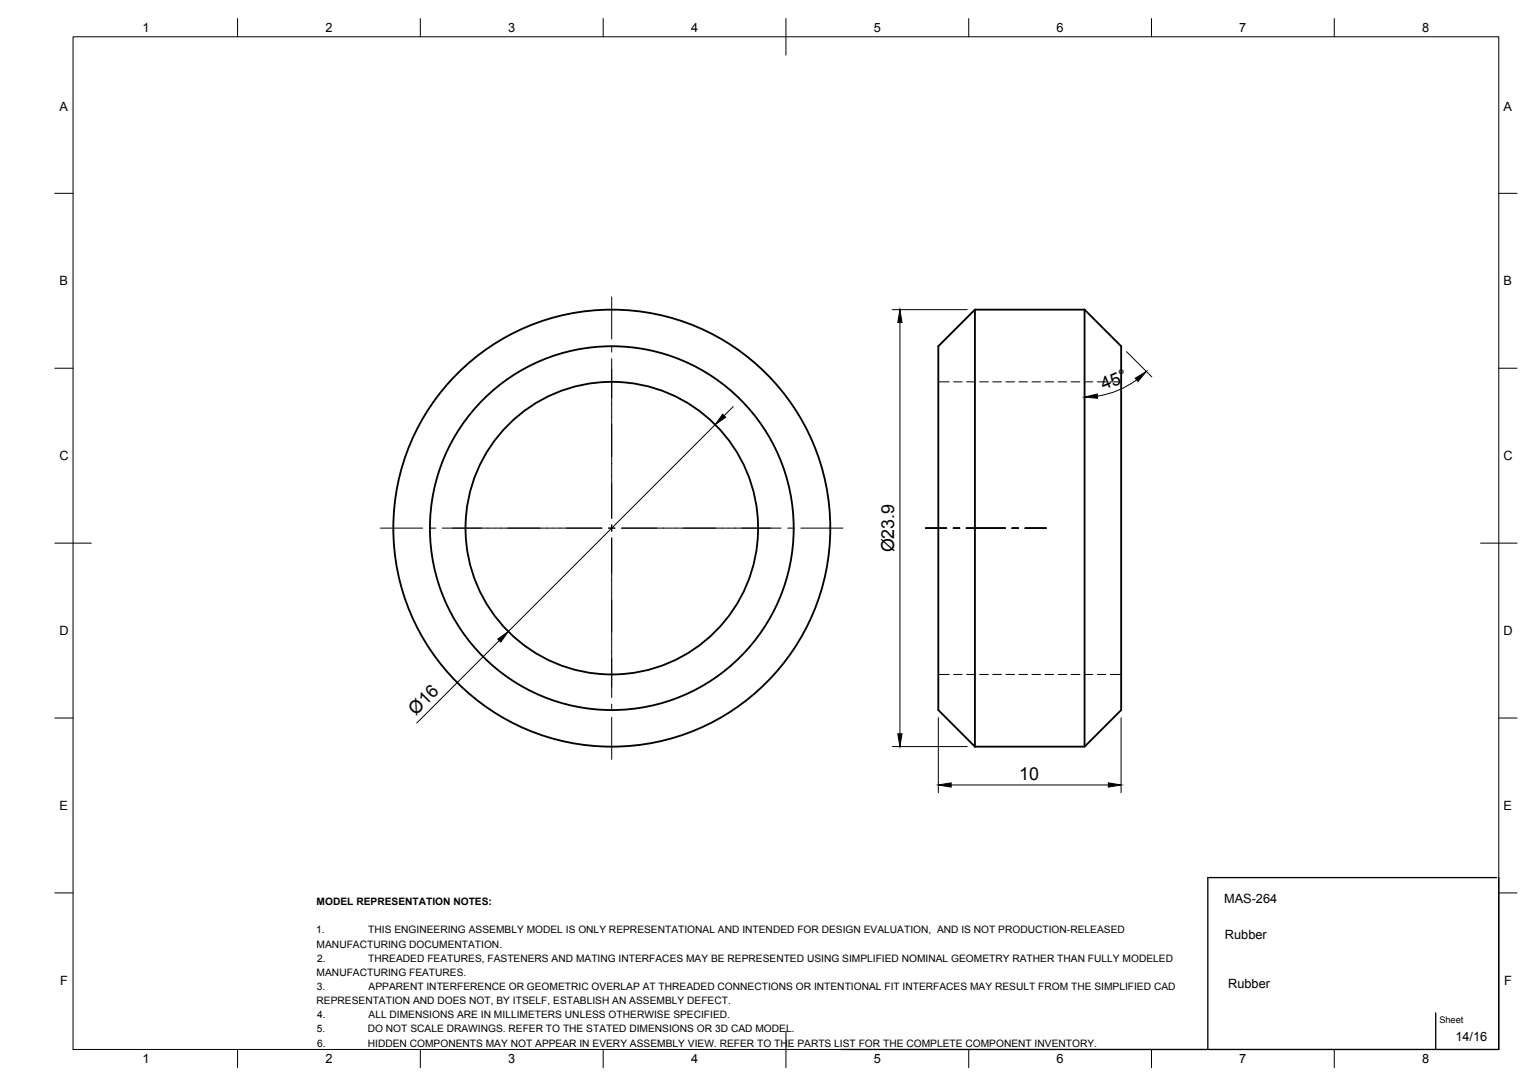
ISO-10303-21;
HEADER;
/* Generated by software containing ST-Developer
 * from STEP Tools, Inc. (www.steptools.com) 
 */

FILE_DESCRIPTION(
/* description */ (''),
/* implementation_level */ '2;1');

FILE_NAME(
/* name */ 'Rubber.step',
/* time_stamp */ '2026-10-12T15:37:13-07:00',
/* author */ (''),
/* organization */ (''),
/* preprocessor_version */ 'ST-DEVELOPER v20.2',
/* originating_system */ 'Autodesk Translation Framework v15.15.0.0',
/* authorisation */ '');

FILE_SCHEMA (('AUTOMOTIVE_DESIGN { 1 0 10303 214 3 1 1 }'));
ENDSEC;

DATA;
#10=MECHANICAL_DESIGN_GEOMETRIC_PRESENTATION_REPRESENTATION('',(#334),#36460);
#107=SHAPE_REPRESENTATION_RELATIONSHIP('SRR','None',#36519,#120);
#120=ADVANCED_BREP_SHAPE_REPRESENTATION('',(#366),#36448);
#159=FACE_BOUND('',#1976,.T.);
#160=FACE_BOUND('',#1979,.T.);
#313=CONICAL_SURFACE('',#11889,10.9505,0.785398163397447);
#314=CONICAL_SURFACE('',#11896,10.9505,0.785398163397447);
#334=STYLED_ITEM('',(#36597),#366);
#366=MANIFOLD_SOLID_BREP('Body1',#11270);
#521=PLANE('',#11894);
#522=PLANE('',#11898);
#1332=FACE_OUTER_BOUND('',#1973,.T.);
#1333=FACE_OUTER_BOUND('',#1974,.T.);
#1334=FACE_OUTER_BOUND('',#1975,.T.);
#1335=FACE_OUTER_BOUND('',#1977,.T.);
#1336=FACE_OUTER_BOUND('',#1978,.T.);
#1337=FACE_OUTER_BOUND('',#1980,.T.);
#1973=EDGE_LOOP('',(#8850,#8851,#8852,#8853));
#1974=EDGE_LOOP('',(#8854,#8855,#8856,#8857));
#1975=EDGE_LOOP('',(#8858));
#1976=EDGE_LOOP('',(#8859));
#1977=EDGE_LOOP('',(#8860,#8861,#8862,#8863));
#1978=EDGE_LOOP('',(#8864));
#1979=EDGE_LOOP('',(#8865));
#1980=EDGE_LOOP('',(#8866,#8867,#8868,#8869));
#2781=LINE('',#34619,#3727);
#2782=LINE('',#34624,#3728);
#2783=LINE('',#34630,#3729);
#2784=LINE('',#34636,#3730);
#3727=VECTOR('',#13736,10.9505);
#3728=VECTOR('',#13743,11.9505);
#3729=VECTOR('',#13750,10.9505);
#3730=VECTOR('',#13759,8.00000000000001);
#4386=CIRCLE('',#11890,11.9505);
#4387=CIRCLE('',#11891,9.95049999999999);
#4388=CIRCLE('',#11893,11.9505);
#4389=CIRCLE('',#11895,8.00000000000001);
#4390=CIRCLE('',#11897,9.95049999999999);
#4391=CIRCLE('',#11899,8.00000000000001);
#5123=VERTEX_POINT('',#34616);
#5124=VERTEX_POINT('',#34618);
#5125=VERTEX_POINT('',#34622);
#5126=VERTEX_POINT('',#34626);
#5127=VERTEX_POINT('',#34629);
#5128=VERTEX_POINT('',#34633);
#6456=EDGE_CURVE('',#5123,#5123,#4386,.T.);
#6457=EDGE_CURVE('',#5123,#5124,#2781,.T.);
#6458=EDGE_CURVE('',#5124,#5124,#4387,.T.);
#6459=EDGE_CURVE('',#5125,#5125,#4388,.T.);
#6460=EDGE_CURVE('',#5125,#5123,#2782,.T.);
#6461=EDGE_CURVE('',#5126,#5126,#4389,.T.);
#6462=EDGE_CURVE('',#5125,#5127,#2783,.T.);
#6463=EDGE_CURVE('',#5127,#5127,#4390,.T.);
#6464=EDGE_CURVE('',#5128,#5128,#4391,.T.);
#6465=EDGE_CURVE('',#5126,#5128,#2784,.T.);
#8850=ORIENTED_EDGE('',*,*,#6456,.T.);
#8851=ORIENTED_EDGE('',*,*,#6457,.T.);
#8852=ORIENTED_EDGE('',*,*,#6458,.T.);
#8853=ORIENTED_EDGE('',*,*,#6457,.F.);
#8854=ORIENTED_EDGE('',*,*,#6459,.F.);
#8855=ORIENTED_EDGE('',*,*,#6460,.T.);
#8856=ORIENTED_EDGE('',*,*,#6456,.F.);
#8857=ORIENTED_EDGE('',*,*,#6460,.F.);
#8858=ORIENTED_EDGE('',*,*,#6458,.F.);
#8859=ORIENTED_EDGE('',*,*,#6461,.T.);
#8860=ORIENTED_EDGE('',*,*,#6459,.T.);
#8861=ORIENTED_EDGE('',*,*,#6462,.T.);
#8862=ORIENTED_EDGE('',*,*,#6463,.T.);
#8863=ORIENTED_EDGE('',*,*,#6462,.F.);
#8864=ORIENTED_EDGE('',*,*,#6463,.F.);
#8865=ORIENTED_EDGE('',*,*,#6464,.T.);
#8866=ORIENTED_EDGE('',*,*,#6461,.F.);
#8867=ORIENTED_EDGE('',*,*,#6465,.T.);
#8868=ORIENTED_EDGE('',*,*,#6464,.F.);
#8869=ORIENTED_EDGE('',*,*,#6465,.F.);
#10560=CYLINDRICAL_SURFACE('',#11892,11.9505);
#10561=CYLINDRICAL_SURFACE('',#11900,8.00000000000001);
#10953=ADVANCED_FACE('',(#1332),#313,.T.);
#10954=ADVANCED_FACE('',(#1333),#10560,.T.);
#10955=ADVANCED_FACE('',(#1334,#159),#521,.F.);
#10956=ADVANCED_FACE('',(#1335),#314,.T.);
#10957=ADVANCED_FACE('',(#1336,#160),#522,.T.);
#10958=ADVANCED_FACE('',(#1337),#10561,.F.);
#11270=CLOSED_SHELL('',(#10953,#10954,#10955,#10956,#10957,#10958));
#11888=AXIS2_PLACEMENT_3D('',#34614,#13730,#13731);
#11889=AXIS2_PLACEMENT_3D('',#34615,#13732,#13733);
#11890=AXIS2_PLACEMENT_3D('',#34617,#13734,#13735);
#11891=AXIS2_PLACEMENT_3D('',#34620,#13737,#13738);
#11892=AXIS2_PLACEMENT_3D('',#34621,#13739,#13740);
#11893=AXIS2_PLACEMENT_3D('',#34623,#13741,#13742);
#11894=AXIS2_PLACEMENT_3D('',#34625,#13744,#13745);
#11895=AXIS2_PLACEMENT_3D('',#34627,#13746,#13747);
#11896=AXIS2_PLACEMENT_3D('',#34628,#13748,#13749);
#11897=AXIS2_PLACEMENT_3D('',#34631,#13751,#13752);
#11898=AXIS2_PLACEMENT_3D('',#34632,#13753,#13754);
#11899=AXIS2_PLACEMENT_3D('',#34634,#13755,#13756);
#11900=AXIS2_PLACEMENT_3D('',#34635,#13757,#13758);
#13730=DIRECTION('axis',(0.,0.,1.));
#13731=DIRECTION('refdir',(1.,0.,0.));
#13732=DIRECTION('center_axis',(-1.,0.,0.));
#13733=DIRECTION('ref_axis',(0.,-1.,0.));
#13734=DIRECTION('center_axis',(1.,0.,2.22044604925031E-16));
#13735=DIRECTION('ref_axis',(0.,-1.,0.));
#13736=DIRECTION('',(0.707106781186548,-0.707106781186547,8.65956056235492E-17));
#13737=DIRECTION('center_axis',(-1.,0.,-2.22044604925031E-16));
#13738=DIRECTION('ref_axis',(0.,-1.,0.));
#13739=DIRECTION('center_axis',(-1.,0.,0.));
#13740=DIRECTION('ref_axis',(0.,-1.,0.));
#13741=DIRECTION('center_axis',(-1.,0.,-2.22044604925031E-16));
#13742=DIRECTION('ref_axis',(0.,-1.,0.));
#13743=DIRECTION('',(1.,0.,0.));
#13744=DIRECTION('center_axis',(-1.,0.,-2.22044604925031E-16));
#13745=DIRECTION('ref_axis',(0.,-1.,0.));
#13746=DIRECTION('center_axis',(-1.,5.47382212626881E-48,-2.22044604925031E-16));
#13747=DIRECTION('ref_axis',(-5.47382212626881E-48,-1.,-1.21543267145725E-63));
#13748=DIRECTION('center_axis',(1.,0.,0.));
#13749=DIRECTION('ref_axis',(0.,-1.,0.));
#13750=DIRECTION('',(-0.707106781186548,-0.707106781186547,-8.65956056235492E-17));
#13751=DIRECTION('center_axis',(1.,0.,2.22044604925031E-16));
#13752=DIRECTION('ref_axis',(0.,-1.,0.));
#13753=DIRECTION('center_axis',(-1.,0.,-2.22044604925031E-16));
#13754=DIRECTION('ref_axis',(0.,-1.,0.));
#13755=DIRECTION('center_axis',(1.,-5.47382212626881E-48,2.22044604925031E-16));
#13756=DIRECTION('ref_axis',(-5.47382212626881E-48,-1.,-1.21543267145725E-63));
#13757=DIRECTION('center_axis',(-1.,0.,0.));
#13758=DIRECTION('ref_axis',(0.,-1.,0.));
#13759=DIRECTION('',(-1.,0.,0.));
#34614=CARTESIAN_POINT('',(0.,0.,0.));
#34615=CARTESIAN_POINT('Origin',(-6.,190.828431883169,20.8299327490105));
#34616=CARTESIAN_POINT('',(-7.,202.778931883169,20.8299327490105));
#34617=CARTESIAN_POINT('Origin',(-7.,190.828431883169,20.8299327490105));
#34618=CARTESIAN_POINT('',(-5.,200.778931883169,20.8299327490105));
#34619=CARTESIAN_POINT('',(-6.,201.778931883169,20.8299327490105));
#34620=CARTESIAN_POINT('Origin',(-5.,190.828431883169,20.8299327490105));
#34621=CARTESIAN_POINT('Origin',(-10.,190.828431883169,20.8299327490105));
#34622=CARTESIAN_POINT('',(-13.,202.778931883169,20.8299327490105));
#34623=CARTESIAN_POINT('Origin',(-13.,190.828431883169,20.8299327490105));
#34624=CARTESIAN_POINT('',(-10.,202.778931883169,20.8299327490105));
#34625=CARTESIAN_POINT('Origin',(-5.,190.828431883169,20.8299327490105));
#34626=CARTESIAN_POINT('',(-5.,198.828431883169,20.8299327490105));
#34627=CARTESIAN_POINT('Origin',(-5.,190.828431883169,20.8299327490105));
#34628=CARTESIAN_POINT('Origin',(-14.,190.828431883169,20.8299327490105));
#34629=CARTESIAN_POINT('',(-15.,200.778931883169,20.8299327490105));
#34630=CARTESIAN_POINT('',(-14.,201.778931883169,20.8299327490105));
#34631=CARTESIAN_POINT('Origin',(-15.,190.828431883169,20.8299327490105));
#34632=CARTESIAN_POINT('Origin',(-15.,190.828431883169,20.8299327490105));
#34633=CARTESIAN_POINT('',(-15.,198.828431883169,20.8299327490105));
#34634=CARTESIAN_POINT('Origin',(-15.,190.828431883169,20.8299327490105));
#34635=CARTESIAN_POINT('Origin',(-10.,190.828431883169,20.8299327490105));
#34636=CARTESIAN_POINT('',(-10.,198.828431883169,20.8299327490105));
#36432=UNCERTAINTY_MEASURE_WITH_UNIT(LENGTH_MEASURE(0.01),#36461,
'DISTANCE_ACCURACY_VALUE',
'Maximum model space distance between geometric entities at asserted c
onnectivities');
#36444=UNCERTAINTY_MEASURE_WITH_UNIT(LENGTH_MEASURE(0.01),#36461,
'DISTANCE_ACCURACY_VALUE',
'Maximum model space distance between geometric entities at asserted c
onnectivities');
#36448=(
GEOMETRIC_REPRESENTATION_CONTEXT(3)
GLOBAL_UNCERTAINTY_ASSIGNED_CONTEXT((#36432))
GLOBAL_UNIT_ASSIGNED_CONTEXT((#36461,#36463,#36464))
REPRESENTATION_CONTEXT('','3D')
);
#36460=(
GEOMETRIC_REPRESENTATION_CONTEXT(3)
GLOBAL_UNCERTAINTY_ASSIGNED_CONTEXT((#36444))
GLOBAL_UNIT_ASSIGNED_CONTEXT((#36461,#36463,#36464))
REPRESENTATION_CONTEXT('','3D')
);
#36461=(
LENGTH_UNIT()
NAMED_UNIT(*)
SI_UNIT(.MILLI.,.METRE.)
);
#36463=(
NAMED_UNIT(*)
PLANE_ANGLE_UNIT()
SI_UNIT($,.RADIAN.)
);
#36464=(
NAMED_UNIT(*)
SI_UNIT($,.STERADIAN.)
SOLID_ANGLE_UNIT()
);
#36468=SHAPE_DEFINITION_REPRESENTATION(#36483,#36519);
#36483=PRODUCT_DEFINITION_SHAPE('',$,#36535);
#36519=SHAPE_REPRESENTATION('',(#11888),#36448);
#36531=PRODUCT_DEFINITION_CONTEXT('part definition',#36578,'design');
#36535=PRODUCT_DEFINITION('Rubber','Rubber',#36550,#36531);
#36550=PRODUCT_DEFINITION_FORMATION('',$,#36583);
#36578=APPLICATION_CONTEXT(
'Core Data for Automotive Mechanical Design Process');
#36579=PRODUCT_CONTEXT('part definition',#36578,'mechanical');
#36583=PRODUCT('Rubber','Rubber',$,(#36579));
#36597=PRESENTATION_STYLE_ASSIGNMENT((#36602));
#36602=SURFACE_STYLE_USAGE(.BOTH.,#36607);
#36607=SURFACE_SIDE_STYLE('',(#36612));
#36612=SURFACE_STYLE_FILL_AREA(#36617);
#36617=FILL_AREA_STYLE('Opaque(39,39,39)',(#36622));
#36622=FILL_AREA_STYLE_COLOUR('Opaque(39,39,39)',#36627);
#36627=COLOUR_RGB('Opaque(39,39,39)', 0.31764706, 0.68627451, 0.89019608);
ENDSEC;
END-ISO-10303-21;
